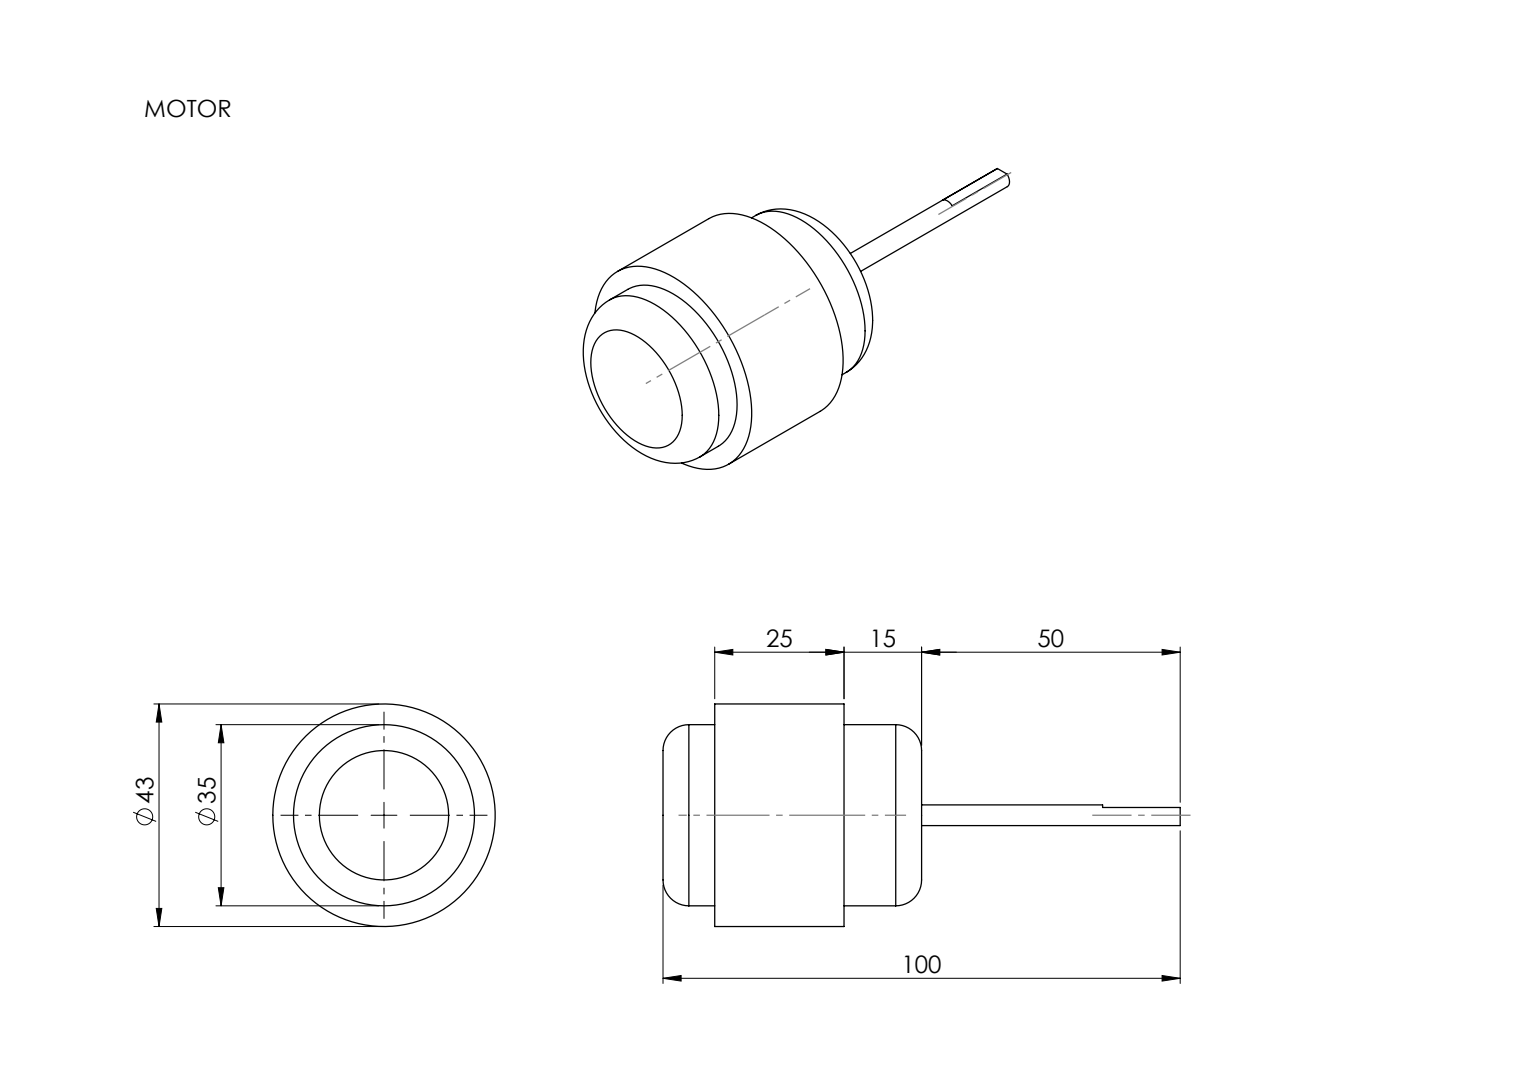
ISO-10303-21;
HEADER;
FILE_DESCRIPTION (('STEP AP214'),
    '1' );
FILE_NAME ('motor.step',
    '2026-10-08T15:02:10',
    ( '' ),
    ( '' ),
    'SwSTEP 2.0',
    'SolidWorks 2026',
    '' );
FILE_SCHEMA (( 'AUTOMOTIVE_DESIGN' ));
ENDSEC;

DATA;
#4=SHAPE_REPRESENTATION_RELATIONSHIP ( 'NONE' , 'NONE' ,  #21505, #10999 ) ;
#67=CARTESIAN_POINT ( 'NONE',  ( 1.322875655532295358, 1.500000000000000000, -105.0000000000000000 ) ) ;
#83=CARTESIAN_POINT ( 'NONE',  ( 12.50000000000000355, 0.000000000000000000, -65.00000000000000000 ) ) ;
#120=CIRCLE ( 'NONE', #7315, 21.50000000000000711 ) ;
#225=AXIS2_PLACEMENT_3D ( 'NONE', #7569, #15900, #3952 ) ;
#288=DIRECTION ( 'NONE',  ( -1.000000000000000000, 0.000000000000000000, 0.000000000000000000 ) ) ;
#339=CARTESIAN_POINT ( 'NONE',  ( 1.322875655532295358, 1.500000000000000000, -120.0000000000000000 ) ) ;
#349=ORIENTED_EDGE ( 'NONE', *, *, #13277, .F. ) ;
#500=CARTESIAN_POINT ( 'NONE',  ( -17.50000000000001066, 2.143131898507869431E-15, -30.00000000000000000 ) ) ;
#540=AXIS2_PLACEMENT_3D ( 'NONE', #11823, #9916, #17115 ) ;
#660=AXIS2_PLACEMENT_3D ( 'NONE', #18313, #757, #9432 ) ;
#665=DIRECTION ( 'NONE',  ( -0.000000000000000000, -0.000000000000000000, -1.000000000000000000 ) ) ;
#686=DIRECTION ( 'NONE',  ( -0.000000000000000000, -0.000000000000000000, -1.000000000000000000 ) ) ;
#711=FACE_OUTER_BOUND ( 'NONE', #8838, .T. ) ;
#756=EDGE_CURVE ( 'NONE', #14896, #1959, #16705, .T. ) ;
#757=DIRECTION ( 'NONE',  ( 0.000000000000000000, 1.000000000000000000, -0.000000000000000000 ) ) ;
#885=CARTESIAN_POINT ( 'NONE',  ( 0.000000000000000000, 0.000000000000000000, -55.00000000000000711 ) ) ;
#907=ORIENTED_EDGE ( 'NONE', *, *, #1716, .T. ) ;
#922=CARTESIAN_POINT ( 'NONE',  ( -21.50000000000000711, 0.000000000000000000, -55.00000000000000711 ) ) ;
#1041=ORIENTED_EDGE ( 'NONE', *, *, #7973, .T. ) ;
#1059=DIRECTION ( 'NONE',  ( -1.000000000000000000, 0.000000000000000000, 0.000000000000000000 ) ) ;
#1102=AXIS2_PLACEMENT_3D ( 'NONE', #16266, #2525, #11420 ) ;
#1133=AXIS2_PLACEMENT_3D ( 'NONE', #4423, #19514, #4101 ) ;
#1161=DIRECTION ( 'NONE',  ( 0.000000000000000000, 0.000000000000000000, 1.000000000000000000 ) ) ;
#1176=PLANE ( 'NONE',  #1102 ) ;
#1275=FACE_OUTER_BOUND ( 'NONE', #18605, .T. ) ;
#1285=CARTESIAN_POINT ( 'NONE',  ( -17.50000000000000355, 2.143131898507868643E-15, -70.00000000000000000 ) ) ;
#1289=CIRCLE ( 'NONE', #225, 21.50000000000000711 ) ;
#1393=ADVANCED_FACE ( 'NONE', ( #19248 ), #3828, .T. ) ;
#1497=AXIS2_PLACEMENT_3D ( 'NONE', #10710, #17575, #21149 ) ;
#1509=EDGE_CURVE ( 'NONE', #11033, #10050, #11370, .T. ) ;
#1518=CARTESIAN_POINT ( 'NONE',  ( -12.50000000000000355, 1.530808498934191916E-15, -25.00000000000000000 ) ) ;
#1534=DIRECTION ( 'NONE',  ( -0.000000000000000000, -0.000000000000000000, -1.000000000000000000 ) ) ;
#1538=CARTESIAN_POINT ( 'NONE',  ( 0.000000000000000000, 0.000000000000000000, -120.0000000000000142 ) ) ;
#1544=AXIS2_PLACEMENT_3D ( 'NONE', #2541, #8986, #15960 ) ;
#1652=( GEOMETRIC_REPRESENTATION_CONTEXT ( 3 ) GLOBAL_UNCERTAINTY_ASSIGNED_CONTEXT ( ( #16412 ) ) GLOBAL_UNIT_ASSIGNED_CONTEXT ( ( #9478, #6196, #11385 ) ) REPRESENTATION_CONTEXT ( 'NONE', 'WORKASPACE' ) );
#1655=DIRECTION ( 'NONE',  ( -1.000000000000000000, 0.000000000000000000, 0.000000000000000000 ) ) ;
#1703=EDGE_LOOP ( 'NONE', ( #10346, #17287, #5811, #6098 ) ) ;
#1716=EDGE_CURVE ( 'NONE', #10973, #3502, #2231, .T. ) ;
#1782=CARTESIAN_POINT ( 'NONE',  ( -17.50000000000000355, 2.143131898507868643E-15, -25.00000000000000000 ) ) ;
#1820=ADVANCED_FACE ( 'NONE', ( #4264 ), #5099, .T. ) ;
#1841=ORIENTED_EDGE ( 'NONE', *, *, #2125, .F. ) ;
#1851=DIRECTION ( 'NONE',  ( 1.000000000000000000, 0.000000000000000000, 0.000000000000000000 ) ) ;
#1889=ORIENTED_EDGE ( 'NONE', *, *, #5608, .T. ) ;
#1954=ORIENTED_EDGE ( 'NONE', *, *, #3358, .F. ) ;
#1959=VERTEX_POINT ( 'NONE', #1782 ) ;
#2125=EDGE_CURVE ( 'NONE', #3502, #10973, #8356, .T. ) ;
#2137=ORIENTED_EDGE ( 'NONE', *, *, #15468, .T. ) ;
#2154=FACE_BOUND ( 'NONE', #18087, .T. ) ;
#2231=CIRCLE ( 'NONE', #4373, 12.50000000000000355 ) ;
#2290=AXIS2_PLACEMENT_3D ( 'NONE', #7537, #2559, #2674 ) ;
#2307=CARTESIAN_POINT ( 'NONE',  ( 17.50000000000000355, 0.000000000000000000, -70.00000000000000000 ) ) ;
#2443=ORIENTED_EDGE ( 'NONE', *, *, #14102, .F. ) ;
#2525=DIRECTION ( 'NONE',  ( 0.000000000000000000, 0.000000000000000000, 1.000000000000000000 ) ) ;
#2541=CARTESIAN_POINT ( 'NONE',  ( 0.000000000000000000, 0.000000000000000000, -70.00000000000000000 ) ) ;
#2559=DIRECTION ( 'NONE',  ( 0.000000000000000000, 0.000000000000000000, -1.000000000000000000 ) ) ;
#2575=DIRECTION ( 'NONE',  ( 0.000000000000000000, 0.000000000000000000, 1.000000000000000000 ) ) ;
#2624=ORIENTED_EDGE ( 'NONE', *, *, #19790, .T. ) ;
#2653=DIRECTION ( 'NONE',  ( -1.000000000000000000, 0.000000000000000000, 0.000000000000000000 ) ) ;
#2674=DIRECTION ( 'NONE',  ( -1.000000000000000000, 0.000000000000000000, 0.000000000000000000 ) ) ;
#2707=DIRECTION ( 'NONE',  ( 1.000000000000000000, 0.000000000000000000, 0.000000000000000000 ) ) ;
#2759=CARTESIAN_POINT ( 'NONE',  ( 0.000000000000000000, 0.000000000000000000, -30.00000000000000000 ) ) ;
#2772=DIRECTION ( 'NONE',  ( 1.000000000000000000, 0.000000000000000000, 0.000000000000000000 ) ) ;
#2801=CIRCLE ( 'NONE', #18270, 17.50000000000001066 ) ;
#2821=AXIS2_PLACEMENT_3D ( 'NONE', #21893, #4675, #16957 ) ;
#2891=DIRECTION ( 'NONE',  ( -0.000000000000000000, -0.000000000000000000, -1.000000000000000000 ) ) ;
#2914=EDGE_CURVE ( 'NONE', #18650, #10973, #5339, .T. ) ;
#2919=AXIS2_PLACEMENT_3D ( 'NONE', #18211, #7637, #2772 ) ;
#2932=VECTOR ( 'NONE', #16594, 1000.000000000000000 ) ;
#2981=ORIENTED_EDGE ( 'NONE', *, *, #8744, .T. ) ;
#3040=VERTEX_POINT ( 'NONE', #16620 ) ;
#3076=MECHANICAL_DESIGN_GEOMETRIC_PRESENTATION_REPRESENTATION('',(#21759),#15681);
#3123=CARTESIAN_POINT ( 'NONE',  ( 0.000000000000000000, 0.000000000000000000, -70.00000000000000000 ) ) ;
#3153=EDGE_LOOP ( 'NONE', ( #14173, #10426, #15370, #5728 ) ) ;
#3180=DIRECTION ( 'NONE',  ( -0.000000000000000000, -0.000000000000000000, -1.000000000000000000 ) ) ;
#3186=ADVANCED_FACE ( 'NONE', ( #16185 ), #18207, .T. ) ;
#3214=DIRECTION ( 'NONE',  ( 1.000000000000000000, 0.000000000000000000, 0.000000000000000000 ) ) ;
#3222=DIRECTION ( 'NONE',  ( -1.000000000000000000, 0.000000000000000000, 0.000000000000000000 ) ) ;
#3358=EDGE_CURVE ( 'NONE', #20674, #9897, #2801, .T. ) ;
#3364=AXIS2_PLACEMENT_3D ( 'NONE', #18542, #13356, #13475 ) ;
#3367=DIRECTION ( 'NONE',  ( -0.000000000000000000, -0.000000000000000000, -1.000000000000000000 ) ) ;
#3437=ORIENTED_EDGE ( 'NONE', *, *, #20358, .F. ) ;
#3438=MECHANICAL_DESIGN_GEOMETRIC_PRESENTATION_REPRESENTATION('',(#17109),#9213);
#3502=VERTEX_POINT ( 'NONE', #9985 ) ;
#3510=CARTESIAN_POINT ( 'NONE',  ( 0.000000000000000000, 0.000000000000000000, -120.0000000000000142 ) ) ;
#3538=ADVANCED_FACE ( 'NONE', ( #22237 ), #13622, .T. ) ;
#3714=LINE ( 'NONE', #4051, #14959 ) ;
#3828=PLANE ( 'NONE',  #1497 ) ;
#3873=VERTEX_POINT ( 'NONE', #67 ) ;
#3879=EDGE_LOOP ( 'NONE', ( #907, #18094 ) ) ;
#3952=DIRECTION ( 'NONE',  ( -1.000000000000000000, 0.000000000000000000, 0.000000000000000000 ) ) ;
#3999=DIRECTION ( 'NONE',  ( -0.000000000000000000, -0.000000000000000000, -1.000000000000000000 ) ) ;
#4051=CARTESIAN_POINT ( 'NONE',  ( -17.50000000000000355, 2.143131898507868643E-15, -70.00000000000000000 ) ) ;
#4073=CIRCLE ( 'NONE', #8401, 5.000000000000004441 ) ;
#4074=FACE_OUTER_BOUND ( 'NONE', #10781, .T. ) ;
#4101=DIRECTION ( 'NONE',  ( 1.000000000000000000, 0.000000000000000000, 0.000000000000000000 ) ) ;
#4185=CARTESIAN_POINT ( 'NONE',  ( -1.322875655532295358, 1.500000000000000000, -378.2244600276337678 ) ) ;
#4205=ORIENTED_EDGE ( 'NONE', *, *, #11174, .F. ) ;
#4264=FACE_OUTER_BOUND ( 'NONE', #16799, .T. ) ;
#4302=LINE ( 'NONE', #4747, #15666 ) ;
#4354=CARTESIAN_POINT ( 'NONE',  ( 0.000000000000000000, 0.000000000000000000, -70.00000000000000000 ) ) ;
#4373=AXIS2_PLACEMENT_3D ( 'NONE', #14970, #4701, #14853 ) ;
#4398=CIRCLE ( 'NONE', #17007, 17.50000000000001066 ) ;
#4423=CARTESIAN_POINT ( 'NONE',  ( 0.000000000000000000, 0.000000000000000000, -70.00000000000000000 ) ) ;
#4469=CARTESIAN_POINT ( 'NONE',  ( 0.000000000000000000, 0.000000000000000000, -105.0000000000000142 ) ) ;
#4499=CARTESIAN_POINT ( 'NONE',  ( 0.000000000000000000, 0.000000000000000000, -70.00000000000000000 ) ) ;
#4512=CARTESIAN_POINT ( 'NONE',  ( 2.000000000000000000, 0.000000000000000000, -120.0000000000000142 ) ) ;
#4528=APPLICATION_CONTEXT ( 'automotive_design' ) ;
#4544=FACE_BOUND ( 'NONE', #13844, .T. ) ;
#4576=ADVANCED_FACE ( 'NONE', ( #7498 ), #14585, .T. ) ;
#4581=CARTESIAN_POINT ( 'NONE',  ( 1.322875655532295358, 1.500000000000000000, -378.2244600276337678 ) ) ;
#4592=ORIENTED_EDGE ( 'NONE', *, *, #6914, .F. ) ;
#4601=EDGE_CURVE ( 'NONE', #11033, #21666, #20906, .T. ) ;
#4675=DIRECTION ( 'NONE',  ( 0.000000000000000000, 0.000000000000000000, 1.000000000000000000 ) ) ;
#4701=DIRECTION ( 'NONE',  ( 0.000000000000000000, 0.000000000000000000, 1.000000000000000000 ) ) ;
#4747=CARTESIAN_POINT ( 'NONE',  ( 21.50000000000001066, 2.632990618166810813E-15, -65.00000000000000000 ) ) ;
#4781=DIRECTION ( 'NONE',  ( -0.000000000000000000, -0.000000000000000000, -1.000000000000000000 ) ) ;
#4838=CARTESIAN_POINT ( 'NONE',  ( 0.000000000000000000, 0.000000000000000000, -30.00000000000000000 ) ) ;
#4919=DIRECTION ( 'NONE',  ( 0.000000000000000000, 0.000000000000000000, -1.000000000000000000 ) ) ;
#4928=EDGE_LOOP ( 'NONE', ( #14011, #17456, #18782, #21763 ) ) ;
#4962=EDGE_CURVE ( 'NONE', #1959, #18650, #20526, .T. ) ;
#4993=ORIENTED_EDGE ( 'NONE', *, *, #12242, .T. ) ;
#5016=ADVANCED_FACE ( 'NONE', ( #8082 ), #9066, .T. ) ;
#5018=FACE_OUTER_BOUND ( 'NONE', #18314, .T. ) ;
#5050=PRODUCT_DEFINITION ( 'UNKNOWN', '', #20347, #14402 ) ;
#5099=TOROIDAL_SURFACE ( 'NONE', #20909, 12.50000000000000355, 5.000000000000000000 ) ;
#5165=AXIS2_PLACEMENT_3D ( 'NONE', #19638, #17970, #9201 ) ;
#5180=CARTESIAN_POINT ( 'NONE',  ( -12.50000000000000355, 1.530808498934191916E-15, -65.00000000000000000 ) ) ;
#5198=CIRCLE ( 'NONE', #540, 17.50000000000000355 ) ;
#5339=CIRCLE ( 'NONE', #13989, 5.000000000000000888 ) ;
#5369=DIRECTION ( 'NONE',  ( 0.000000000000000000, 0.000000000000000000, 1.000000000000000000 ) ) ;
#5498=DIRECTION ( 'NONE',  ( -0.000000000000000000, -0.000000000000000000, 1.000000000000000000 ) ) ;
#5545=ADVANCED_FACE ( 'NONE', ( #5018 ), #6604, .T. ) ;
#5550=ORIENTED_EDGE ( 'NONE', *, *, #17171, .F. ) ;
#5552=ORIENTED_EDGE ( 'NONE', *, *, #15025, .F. ) ;
#5608=EDGE_CURVE ( 'NONE', #7196, #9986, #6530, .T. ) ;
#5692=CARTESIAN_POINT ( 'NONE',  ( -1.322875655532295136, 1.500000000000000000, -120.0000000000000142 ) ) ;
#5728=ORIENTED_EDGE ( 'NONE', *, *, #2914, .F. ) ;
#5750=( NAMED_UNIT ( * ) PLANE_ANGLE_UNIT ( ) SI_UNIT ( $, .RADIAN. ) );
#5781=EDGE_LOOP ( 'NONE', ( #20629, #3437, #20188, #5552 ) ) ;
#5811=ORIENTED_EDGE ( 'NONE', *, *, #6066, .T. ) ;
#5833=DIRECTION ( 'NONE',  ( 1.000000000000000000, 0.000000000000000000, 0.000000000000000000 ) ) ;
#6066=EDGE_CURVE ( 'NONE', #13719, #18650, #19408, .T. ) ;
#6098=ORIENTED_EDGE ( 'NONE', *, *, #13277, .T. ) ;
#6180=ADVANCED_FACE ( 'NONE', ( #4544, #18180 ), #1176, .F. ) ;
#6181=AXIS2_PLACEMENT_3D ( 'NONE', #14396, #5369, #21015 ) ;
#6194=CIRCLE ( 'NONE', #10881, 2.000000000000000000 ) ;
#6196=( NAMED_UNIT ( * ) PLANE_ANGLE_UNIT ( ) SI_UNIT ( $, .RADIAN. ) );
#6203=CARTESIAN_POINT ( 'NONE',  ( 17.50000000000001066, 0.000000000000000000, -55.00000000000000711 ) ) ;
#6225=AXIS2_PLACEMENT_3D ( 'NONE', #11498, #16348, #19926 ) ;
#6287=ORIENTED_EDGE ( 'NONE', *, *, #17683, .F. ) ;
#6414=DIRECTION ( 'NONE',  ( 1.000000000000000000, 0.000000000000000000, 0.000000000000000000 ) ) ;
#6454=EDGE_CURVE ( 'NONE', #14043, #20674, #3714, .T. ) ;
#6524=CARTESIAN_POINT ( 'NONE',  ( 17.50000000000000355, 0.000000000000000000, -25.00000000000000000 ) ) ;
#6530=CIRCLE ( 'NONE', #9416, 2.000000000000000000 ) ;
#6532=( NAMED_UNIT ( * ) SI_UNIT ( $, .STERADIAN. ) SOLID_ANGLE_UNIT ( ) );
#6604=CYLINDRICAL_SURFACE ( 'NONE', #19110, 17.50000000000000355 ) ;
#6650=PRESENTATION_STYLE_ASSIGNMENT (( #18694 ) ) ;
#6669=ORIENTED_EDGE ( 'NONE', *, *, #13487, .T. ) ;
#6677=AXIS2_PLACEMENT_3D ( 'NONE', #18028, #16226, #2707 ) ;
#6692=COLOUR_RGB ( '', 0.66274510, 0.83137255, 0.94901961) ;
#6748=ORIENTED_EDGE ( 'NONE', *, *, #756, .T. ) ;
#6764=( LENGTH_UNIT ( ) NAMED_UNIT ( * ) SI_UNIT ( .MILLI., .METRE. ) );
#6914=EDGE_CURVE ( 'NONE', #9939, #9897, #16068, .T. ) ;
#7196=VERTEX_POINT ( 'NONE', #19369 ) ;
#7207=DIRECTION ( 'NONE',  ( -1.000000000000000000, 0.000000000000000000, 0.000000000000000000 ) ) ;
#7261=VECTOR ( 'NONE', #10925, 1000.000000000000000 ) ;
#7291=DIRECTION ( 'NONE',  ( 1.000000000000000000, 0.000000000000000000, 0.000000000000000000 ) ) ;
#7315=AXIS2_PLACEMENT_3D ( 'NONE', #885, #665, #16199 ) ;
#7318=CARTESIAN_POINT ( 'NONE',  ( 0.000000000000000000, 0.000000000000000000, -120.0000000000000142 ) ) ;
#7335=ADVANCED_FACE ( 'NONE', ( #12628, #2154 ), #9034, .F. ) ;
#7352=DIRECTION ( 'NONE',  ( -0.000000000000000000, 0.000000000000000000, -1.000000000000000000 ) ) ;
#7376=AXIS2_PLACEMENT_3D ( 'NONE', #1518, #20408, #8723 ) ;
#7396=AXIS2_PLACEMENT_3D ( 'NONE', #15532, #3367, #10249 ) ;
#7414=VECTOR ( 'NONE', #17361, 1000.000000000000000 ) ;
#7421=ORIENTED_EDGE ( 'NONE', *, *, #8542, .F. ) ;
#7498=FACE_OUTER_BOUND ( 'NONE', #1703, .T. ) ;
#7537=CARTESIAN_POINT ( 'NONE',  ( 0.000000000000000000, 0.000000000000000000, -105.0000000000000142 ) ) ;
#7540=DIRECTION ( 'NONE',  ( 0.000000000000000000, 0.000000000000000000, 1.000000000000000000 ) ) ;
#7569=CARTESIAN_POINT ( 'NONE',  ( 0.000000000000000000, 0.000000000000000000, -55.00000000000000711 ) ) ;
#7612=ORIENTED_EDGE ( 'NONE', *, *, #3358, .T. ) ;
#7637=DIRECTION ( 'NONE',  ( 0.000000000000000000, 0.000000000000000000, 1.000000000000000000 ) ) ;
#7673=AXIS2_PLACEMENT_3D ( 'NONE', #9084, #3999, #7291 ) ;
#7728=DIRECTION ( 'NONE',  ( -0.000000000000000000, -0.000000000000000000, -1.000000000000000000 ) ) ;
#7862=UNCERTAINTY_MEASURE_WITH_UNIT (LENGTH_MEASURE( 1.000000000000000082E-05 ), #6764, 'distance_accuracy_value', 'NONE');
#7942=ORIENTED_EDGE ( 'NONE', *, *, #9134, .T. ) ;
#7973=EDGE_CURVE ( 'NONE', #14896, #13719, #8140, .T. ) ;
#8042=AXIS2_PLACEMENT_3D ( 'NONE', #7318, #5498, #19229 ) ;
#8082=FACE_OUTER_BOUND ( 'NONE', #5781, .T. ) ;
#8131=VECTOR ( 'NONE', #21323, 1000.000000000000000 ) ;
#8140=CIRCLE ( 'NONE', #20705, 17.50000000000001066 ) ;
#8159=DIRECTION ( 'NONE',  ( 0.000000000000000000, 0.000000000000000000, 1.000000000000000000 ) ) ;
#8297=APPLICATION_CONTEXT ( 'automotive_design' ) ;
#8350=VERTEX_POINT ( 'NONE', #17645 ) ;
#8356=CIRCLE ( 'NONE', #6181, 12.50000000000000355 ) ;
#8385=DIRECTION ( 'NONE',  ( 0.000000000000000000, 0.000000000000000000, -1.000000000000000000 ) ) ;
#8396=CARTESIAN_POINT ( 'NONE',  ( -2.000000000000000000, 2.449293598294706414E-16, -120.0000000000000142 ) ) ;
#8401=AXIS2_PLACEMENT_3D ( 'NONE', #83, #12016, #4919 ) ;
#8416=DIRECTION ( 'NONE',  ( 0.000000000000000000, 0.000000000000000000, -1.000000000000000000 ) ) ;
#8449=ADVANCED_FACE ( 'NONE', ( #12579, #17871 ), #19422, .F. ) ;
#8482=ORIENTED_EDGE ( 'NONE', *, *, #4601, .T. ) ;
#8534=PRODUCT_DEFINITION_SHAPE ( 'NONE', 'NONE',  #5050 ) ;
#8542=EDGE_CURVE ( 'NONE', #14013, #9212, #19535, .T. ) ;
#8598=FACE_OUTER_BOUND ( 'NONE', #19239, .T. ) ;
#8691=ORIENTED_EDGE ( 'NONE', *, *, #21072, .T. ) ;
#8723=DIRECTION ( 'NONE',  ( -1.000000000000000000, 1.224646799147353454E-16, 0.000000000000000000 ) ) ;
#8735=CIRCLE ( 'NONE', #17733, 12.50000000000000355 ) ;
#8744=EDGE_CURVE ( 'NONE', #13719, #14896, #4398, .T. ) ;
#8783=EDGE_CURVE ( 'NONE', #21666, #11033, #11954, .T. ) ;
#8789=CIRCLE ( 'NONE', #18130, 17.50000000000000355 ) ;
#8838=EDGE_LOOP ( 'NONE', ( #4205, #13568, #21735, #16900, #15673, #4993, #9825, #16082 ) ) ;
#8874=CARTESIAN_POINT ( 'NONE',  ( 2.000000000000000000, 0.000000000000000000, -70.00000000000000000 ) ) ;
#8986=DIRECTION ( 'NONE',  ( 0.000000000000000000, 0.000000000000000000, 1.000000000000000000 ) ) ;
#9034=PLANE ( 'NONE',  #12451 ) ;
#9066=TOROIDAL_SURFACE ( 'NONE', #2919, 12.50000000000000355, 5.000000000000000000 ) ;
#9084=CARTESIAN_POINT ( 'NONE',  ( 0.000000000000000000, 0.000000000000000000, -70.00000000000000000 ) ) ;
#9096=ORIENTED_EDGE ( 'NONE', *, *, #7973, .F. ) ;
#9127=ORIENTED_EDGE ( 'NONE', *, *, #2914, .T. ) ;
#9134=EDGE_CURVE ( 'NONE', #9986, #14013, #18790, .T. ) ;
#9178=CARTESIAN_POINT ( 'NONE',  ( -17.50000000000001066, 2.143131898507869431E-15, -55.00000000000000711 ) ) ;
#9201=DIRECTION ( 'NONE',  ( 1.000000000000000000, 0.000000000000000000, 0.000000000000000000 ) ) ;
#9212=VERTEX_POINT ( 'NONE', #19049 ) ;
#9213=( GEOMETRIC_REPRESENTATION_CONTEXT ( 3 ) GLOBAL_UNCERTAINTY_ASSIGNED_CONTEXT ( ( #7862 ) ) GLOBAL_UNIT_ASSIGNED_CONTEXT ( ( #6764, #15434, #6532 ) ) REPRESENTATION_CONTEXT ( 'NONE', 'WORKASPACE' ) );
#9260=ADVANCED_FACE ( 'NONE', ( #4074 ), #15801, .T. ) ;
#9320=ORIENTED_EDGE ( 'NONE', *, *, #22019, .F. ) ;
#9360=ORIENTED_EDGE ( 'NONE', *, *, #4962, .T. ) ;
#9393=ORIENTED_EDGE ( 'NONE', *, *, #1509, .F. ) ;
#9403=EDGE_CURVE ( 'NONE', #13305, #8350, #21065, .T. ) ;
#9416=AXIS2_PLACEMENT_3D ( 'NONE', #1538, #8416, #1655 ) ;
#9432=DIRECTION ( 'NONE',  ( 0.000000000000000000, 0.000000000000000000, 1.000000000000000000 ) ) ;
#9448=FACE_OUTER_BOUND ( 'NONE', #15163, .T. ) ;
#9478=( LENGTH_UNIT ( ) NAMED_UNIT ( * ) SI_UNIT ( .MILLI., .METRE. ) );
#9485=VECTOR ( 'NONE', #11457, 1000.000000000000000 ) ;
#9486=CYLINDRICAL_SURFACE ( 'NONE', #6225, 21.50000000000001066 ) ;
#9655=CARTESIAN_POINT ( 'NONE',  ( 12.50000000000000355, 0.000000000000000000, -20.00000000000000000 ) ) ;
#9737=ORIENTED_EDGE ( 'NONE', *, *, #6454, .F. ) ;
#9803=AXIS2_PLACEMENT_3D ( 'NONE', #12905, #4781, #2653 ) ;
#9825=ORIENTED_EDGE ( 'NONE', *, *, #12429, .F. ) ;
#9870=ORIENTED_EDGE ( 'NONE', *, *, #20358, .T. ) ;
#9897=VERTEX_POINT ( 'NONE', #6203 ) ;
#9916=DIRECTION ( 'NONE',  ( 0.000000000000000000, 0.000000000000000000, 1.000000000000000000 ) ) ;
#9939=VERTEX_POINT ( 'NONE', #19811 ) ;
#9983=ADVANCED_FACE ( 'NONE', ( #14885 ), #9486, .T. ) ;
#9985=CARTESIAN_POINT ( 'NONE',  ( -12.50000000000000355, 1.836970198721030378E-15, -20.00000000000000000 ) ) ;
#9986=VERTEX_POINT ( 'NONE', #4512 ) ;
#10050=VERTEX_POINT ( 'NONE', #922 ) ;
#10066=CARTESIAN_POINT ( 'NONE',  ( 0.000000000000000000, 0.000000000000000000, -120.0000000000000142 ) ) ;
#10120=ORIENTED_EDGE ( 'NONE', *, *, #10180, .T. ) ;
#10124=ORIENTED_EDGE ( 'NONE', *, *, #21072, .F. ) ;
#10153=DIRECTION ( 'NONE',  ( 1.224646799147353207E-16, 1.000000000000000000, -0.000000000000000000 ) ) ;
#10180=EDGE_CURVE ( 'NONE', #3040, #14043, #14854, .T. ) ;
#10249=DIRECTION ( 'NONE',  ( -1.000000000000000000, 0.000000000000000000, 0.000000000000000000 ) ) ;
#10346=ORIENTED_EDGE ( 'NONE', *, *, #756, .F. ) ;
#10367=ORIENTED_EDGE ( 'NONE', *, *, #15468, .F. ) ;
#10390=DIRECTION ( 'NONE',  ( 0.000000000000000000, 0.000000000000000000, -1.000000000000000000 ) ) ;
#10416=CYLINDRICAL_SURFACE ( 'NONE', #11251, 21.50000000000001066 ) ;
#10426=ORIENTED_EDGE ( 'NONE', *, *, #14102, .T. ) ;
#10548=VECTOR ( 'NONE', #3222, 1000.000000000000000 ) ;
#10556=DIRECTION ( 'NONE',  ( -1.000000000000000000, 0.000000000000000000, 0.000000000000000000 ) ) ;
#10610=DIRECTION ( 'NONE',  ( -1.000000000000000000, 0.000000000000000000, -0.000000000000000000 ) ) ;
#10685=EDGE_LOOP ( 'NONE', ( #9870, #19241 ) ) ;
#10710=CARTESIAN_POINT ( 'NONE',  ( 0.000000000000000000, 0.000000000000000000, -20.00000000000000000 ) ) ;
#10724=PRESENTATION_STYLE_ASSIGNMENT (( #17813 ) ) ;
#10740=ORIENTED_EDGE ( 'NONE', *, *, #13487, .F. ) ;
#10781=EDGE_LOOP ( 'NONE', ( #9737, #19755, #12772, #2137 ) ) ;
#10881=AXIS2_PLACEMENT_3D ( 'NONE', #4499, #686, #14429 ) ;
#10925=DIRECTION ( 'NONE',  ( -0.000000000000000000, -0.000000000000000000, -1.000000000000000000 ) ) ;
#10927=AXIS2_PLACEMENT_3D ( 'NONE', #4469, #11350, #18220 ) ;
#10973=VERTEX_POINT ( 'NONE', #9655 ) ;
#10979=CARTESIAN_POINT ( 'NONE',  ( 0.000000000000000000, 0.000000000000000000, -30.00000000000000000 ) ) ;
#10999=ADVANCED_BREP_SHAPE_REPRESENTATION ( '', ( #22038, #6677 ), #1652 ) ;
#11013=ORIENTED_EDGE ( 'NONE', *, *, #16421, .F. ) ;
#11025=CARTESIAN_POINT ( 'NONE',  ( 12.50000000000000355, 0.000000000000000000, -70.00000000000000000 ) ) ;
#11033=VERTEX_POINT ( 'NONE', #18319 ) ;
#11174=EDGE_CURVE ( 'NONE', #14013, #13305, #16660, .T. ) ;
#11177=EDGE_LOOP ( 'NONE', ( #17966, #13696 ) ) ;
#11250=CARTESIAN_POINT ( 'NONE',  ( 0.000000000000000000, 0.000000000000000000, -65.00000000000000000 ) ) ;
#11251=AXIS2_PLACEMENT_3D ( 'NONE', #15075, #19067, #288 ) ;
#11330=EDGE_LOOP ( 'NONE', ( #7421, #18893, #17633, #15312 ) ) ;
#11350=DIRECTION ( 'NONE',  ( 0.000000000000000000, 0.000000000000000000, -1.000000000000000000 ) ) ;
#11370=LINE ( 'NONE', #17907, #7261 ) ;
#11385=( NAMED_UNIT ( * ) SI_UNIT ( $, .STERADIAN. ) SOLID_ANGLE_UNIT ( ) );
#11398=EDGE_LOOP ( 'NONE', ( #10124, #17672, #19566, #9320 ) ) ;
#11420=DIRECTION ( 'NONE',  ( 1.000000000000000000, 0.000000000000000000, -0.000000000000000000 ) ) ;
#11429=CARTESIAN_POINT ( 'NONE',  ( -17.50000000000000355, 2.143131898507868643E-15, -65.00000000000000000 ) ) ;
#11457=DIRECTION ( 'NONE',  ( 0.000000000000000000, 0.000000000000000000, 1.000000000000000000 ) ) ;
#11498=CARTESIAN_POINT ( 'NONE',  ( 0.000000000000000000, 0.000000000000000000, -65.00000000000000000 ) ) ;
#11557=DIRECTION ( 'NONE',  ( 0.000000000000000000, 0.000000000000000000, 1.000000000000000000 ) ) ;
#11568=FACE_OUTER_BOUND ( 'NONE', #11398, .T. ) ;
#11714=DIRECTION ( 'NONE',  ( -0.000000000000000000, -0.000000000000000000, -1.000000000000000000 ) ) ;
#11787=CARTESIAN_POINT ( 'NONE',  ( 0.000000000000000000, 0.000000000000000000, -70.00000000000000000 ) ) ;
#11823=CARTESIAN_POINT ( 'NONE',  ( 0.000000000000000000, 0.000000000000000000, -65.00000000000000000 ) ) ;
#11879=EDGE_CURVE ( 'NONE', #7196, #13305, #15977, .T. ) ;
#11908=ADVANCED_FACE ( 'NONE', ( #14188 ), #14073, .T. ) ;
#11926=VECTOR ( 'NONE', #8159, 1000.000000000000000 ) ;
#11954=CIRCLE ( 'NONE', #9803, 21.50000000000001066 ) ;
#11989=VECTOR ( 'NONE', #7207, 1000.000000000000000 ) ;
#11997=ORIENTED_EDGE ( 'NONE', *, *, #17120, .T. ) ;
#12009=CIRCLE ( 'NONE', #2290, 2.000000000000000000 ) ;
#12016=DIRECTION ( 'NONE',  ( 0.000000000000000000, -1.000000000000000000, 0.000000000000000000 ) ) ;
#12030=CIRCLE ( 'NONE', #7376, 5.000000000000000888 ) ;
#12079=PLANE ( 'NONE',  #20689 ) ;
#12174=CLOSED_SHELL ( 'NONE', ( #5545, #3538, #9983, #14561, #1820, #21092, #9260, #8449, #5016, #11908, #21845, #3186, #12520, #7335, #20015, #6180, #1393, #16205, #4576 ) ) ;
#12242=EDGE_CURVE ( 'NONE', #7196, #3873, #12820, .T. ) ;
#12296=( LENGTH_UNIT ( ) NAMED_UNIT ( * ) SI_UNIT ( .MILLI., .METRE. ) );
#12304=DIRECTION ( 'NONE',  ( 1.000000000000000000, 0.000000000000000000, 0.000000000000000000 ) ) ;
#12412=FILL_AREA_STYLE ('',( #14109 ) ) ;
#12429=EDGE_CURVE ( 'NONE', #8350, #3873, #12009, .T. ) ;
#12451=AXIS2_PLACEMENT_3D ( 'NONE', #15898, #7352, #21054 ) ;
#12520=ADVANCED_FACE ( 'NONE', ( #16418 ), #21684, .T. ) ;
#12530=DIRECTION ( 'NONE',  ( 0.000000000000000000, 0.000000000000000000, 1.000000000000000000 ) ) ;
#12579=FACE_BOUND ( 'NONE', #15188, .T. ) ;
#12628=FACE_OUTER_BOUND ( 'NONE', #11177, .T. ) ;
#12630=( NAMED_UNIT ( * ) SI_UNIT ( $, .STERADIAN. ) SOLID_ANGLE_UNIT ( ) );
#12673=PRODUCT_CONTEXT ( 'NONE', #4528, 'mechanical' ) ;
#12772=ORIENTED_EDGE ( 'NONE', *, *, #6914, .T. ) ;
#12820=LINE ( 'NONE', #4581, #9485 ) ;
#12905=CARTESIAN_POINT ( 'NONE',  ( 0.000000000000000000, 0.000000000000000000, -30.00000000000000000 ) ) ;
#13050=VECTOR ( 'NONE', #14493, 1000.000000000000000 ) ;
#13277=EDGE_CURVE ( 'NONE', #18650, #1959, #8789, .T. ) ;
#13295=ORIENTED_EDGE ( 'NONE', *, *, #11879, .F. ) ;
#13305=VERTEX_POINT ( 'NONE', #5692 ) ;
#13313=DIRECTION ( 'NONE',  ( 1.000000000000000000, 0.000000000000000000, 0.000000000000000000 ) ) ;
#13343=DIRECTION ( 'NONE',  ( -0.000000000000000000, -0.000000000000000000, -1.000000000000000000 ) ) ;
#13356=DIRECTION ( 'NONE',  ( 0.000000000000000000, 0.000000000000000000, -1.000000000000000000 ) ) ;
#13398=VECTOR ( 'NONE', #12530, 1000.000000000000000 ) ;
#13475=DIRECTION ( 'NONE',  ( -1.000000000000000000, 0.000000000000000000, 0.000000000000000000 ) ) ;
#13487=EDGE_CURVE ( 'NONE', #9939, #14043, #14889, .T. ) ;
#13551=CARTESIAN_POINT ( 'NONE',  ( 21.50000000000001066, 2.632990618166810813E-15, -30.00000000000000000 ) ) ;
#13559=CARTESIAN_POINT ( 'NONE',  ( 0.000000000000000000, 0.000000000000000000, -25.00000000000000000 ) ) ;
#13568=ORIENTED_EDGE ( 'NONE', *, *, #8542, .T. ) ;
#13622=TOROIDAL_SURFACE ( 'NONE', #2821, 12.50000000000000355, 5.000000000000000000 ) ;
#13696=ORIENTED_EDGE ( 'NONE', *, *, #8783, .F. ) ;
#13719=VERTEX_POINT ( 'NONE', #21653 ) ;
#13745=SURFACE_SIDE_STYLE ('',( #20359 ) ) ;
#13841=AXIS2_PLACEMENT_3D ( 'NONE', #21824, #16664, #6414 ) ;
#13844=EDGE_LOOP ( 'NONE', ( #10367, #1954 ) ) ;
#13936=LINE ( 'NONE', #15401, #10548 ) ;
#13978=DIRECTION ( 'NONE',  ( 1.000000000000000000, 0.000000000000000000, 0.000000000000000000 ) ) ;
#13989=AXIS2_PLACEMENT_3D ( 'NONE', #19653, #16404, #14827 ) ;
#14011=ORIENTED_EDGE ( 'NONE', *, *, #12242, .F. ) ;
#14013=VERTEX_POINT ( 'NONE', #8396 ) ;
#14043=VERTEX_POINT ( 'NONE', #11429 ) ;
#14073=CYLINDRICAL_SURFACE ( 'NONE', #8042, 2.000000000000000000 ) ;
#14102=EDGE_CURVE ( 'NONE', #1959, #3502, #12030, .T. ) ;
#14109=FILL_AREA_STYLE_COLOUR ( '', #6692 ) ;
#14173=ORIENTED_EDGE ( 'NONE', *, *, #4962, .F. ) ;
#14188=FACE_OUTER_BOUND ( 'NONE', #11330, .T. ) ;
#14230=CARTESIAN_POINT ( 'NONE',  ( 0.000000000000000000, 0.000000000000000000, -70.00000000000000000 ) ) ;
#14239=COLOUR_RGB ( '', 0.66274510, 0.83137255, 0.94901961) ;
#14375=EDGE_LOOP ( 'NONE', ( #8482, #8691, #14397, #9393 ) ) ;
#14382=CARTESIAN_POINT ( 'NONE',  ( 17.50000000000000355, 0.000000000000000000, -70.00000000000000000 ) ) ;
#14396=CARTESIAN_POINT ( 'NONE',  ( 0.000000000000000000, 0.000000000000000000, -20.00000000000000000 ) ) ;
#14397=ORIENTED_EDGE ( 'NONE', *, *, #19790, .F. ) ;
#14402=PRODUCT_DEFINITION_CONTEXT ( 'detailed design', #8297, 'design' ) ;
#14429=DIRECTION ( 'NONE',  ( 1.000000000000000000, 0.000000000000000000, 0.000000000000000000 ) ) ;
#14493=DIRECTION ( 'NONE',  ( -0.000000000000000000, -0.000000000000000000, 1.000000000000000000 ) ) ;
#14561=ADVANCED_FACE ( 'NONE', ( #711 ), #16139, .T. ) ;
#14585=CYLINDRICAL_SURFACE ( 'NONE', #1133, 17.50000000000000355 ) ;
#14591=AXIS2_PLACEMENT_3D ( 'NONE', #21744, #1161, #13313 ) ;
#14744=DIRECTION ( 'NONE',  ( 1.000000000000000000, 0.000000000000000000, 0.000000000000000000 ) ) ;
#14827=DIRECTION ( 'NONE',  ( 0.000000000000000000, 0.000000000000000000, -1.000000000000000000 ) ) ;
#14853=DIRECTION ( 'NONE',  ( 1.000000000000000000, 0.000000000000000000, 0.000000000000000000 ) ) ;
#14854=CIRCLE ( 'NONE', #17731, 5.000000000000000888 ) ;
#14885=FACE_OUTER_BOUND ( 'NONE', #14375, .T. ) ;
#14889=CIRCLE ( 'NONE', #5165, 17.50000000000000355 ) ;
#14896=VERTEX_POINT ( 'NONE', #500 ) ;
#14903=CYLINDRICAL_SURFACE ( 'NONE', #14591, 17.50000000000000355 ) ;
#14945=CIRCLE ( 'NONE', #7396, 17.50000000000001066 ) ;
#14959=VECTOR ( 'NONE', #11557, 1000.000000000000000 ) ;
#14970=CARTESIAN_POINT ( 'NONE',  ( 0.000000000000000000, 0.000000000000000000, -20.00000000000000000 ) ) ;
#15025=EDGE_CURVE ( 'NONE', #14043, #9939, #5198, .T. ) ;
#15075=CARTESIAN_POINT ( 'NONE',  ( 0.000000000000000000, 0.000000000000000000, -65.00000000000000000 ) ) ;
#15163=EDGE_LOOP ( 'NONE', ( #2443, #349, #9127, #1841 ) ) ;
#15188=EDGE_LOOP ( 'NONE', ( #11013, #20923 ) ) ;
#15312=ORIENTED_EDGE ( 'NONE', *, *, #16421, .T. ) ;
#15370=ORIENTED_EDGE ( 'NONE', *, *, #1716, .F. ) ;
#15401=CARTESIAN_POINT ( 'NONE',  ( 1.322875655532295358, 1.500000000000000000, -104.9999999999999858 ) ) ;
#15416=ORIENTED_EDGE ( 'NONE', *, *, #6454, .T. ) ;
#15434=( NAMED_UNIT ( * ) PLANE_ANGLE_UNIT ( ) SI_UNIT ( $, .RADIAN. ) );
#15468=EDGE_CURVE ( 'NONE', #9897, #20674, #14945, .T. ) ;
#15532=CARTESIAN_POINT ( 'NONE',  ( 0.000000000000000000, 0.000000000000000000, -55.00000000000000711 ) ) ;
#15646=TOROIDAL_SURFACE ( 'NONE', #17446, 12.50000000000000355, 5.000000000000000000 ) ;
#15666=VECTOR ( 'NONE', #20154, 1000.000000000000000 ) ;
#15673=ORIENTED_EDGE ( 'NONE', *, *, #5608, .F. ) ;
#15681=( GEOMETRIC_REPRESENTATION_CONTEXT ( 3 ) GLOBAL_UNCERTAINTY_ASSIGNED_CONTEXT ( ( #20200 ) ) GLOBAL_UNIT_ASSIGNED_CONTEXT ( ( #12296, #5750, #12630 ) ) REPRESENTATION_CONTEXT ( 'NONE', 'WORKASPACE' ) );
#15801=CYLINDRICAL_SURFACE ( 'NONE', #18432, 17.50000000000000355 ) ;
#15898=CARTESIAN_POINT ( 'NONE',  ( 0.000000000000000000, -17.50000000000001066, -30.00000000000000000 ) ) ;
#15900=DIRECTION ( 'NONE',  ( -0.000000000000000000, -0.000000000000000000, -1.000000000000000000 ) ) ;
#15960=DIRECTION ( 'NONE',  ( 1.000000000000000000, 0.000000000000000000, -0.000000000000000000 ) ) ;
#15977=LINE ( 'NONE', #339, #11989 ) ;
#16065=CARTESIAN_POINT ( 'NONE',  ( 0.000000000000000000, 0.000000000000000000, -25.00000000000000000 ) ) ;
#16068=LINE ( 'NONE', #14382, #8131 ) ;
#16082=ORIENTED_EDGE ( 'NONE', *, *, #9403, .F. ) ;
#16139=CYLINDRICAL_SURFACE ( 'NONE', #13841, 2.000000000000000000 ) ;
#16185=FACE_OUTER_BOUND ( 'NONE', #4928, .T. ) ;
#16199=DIRECTION ( 'NONE',  ( -1.000000000000000000, 0.000000000000000000, 0.000000000000000000 ) ) ;
#16205=ADVANCED_FACE ( 'NONE', ( #9448 ), #15646, .T. ) ;
#16226=DIRECTION ( 'NONE',  ( 0.000000000000000000, 0.000000000000000000, 1.000000000000000000 ) ) ;
#16266=CARTESIAN_POINT ( 'NONE',  ( 0.000000000000000000, -17.50000000000001066, -55.00000000000000711 ) ) ;
#16308=DIRECTION ( 'NONE',  ( 1.000000000000000000, 0.000000000000000000, 0.000000000000000000 ) ) ;
#16348=DIRECTION ( 'NONE',  ( -0.000000000000000000, -0.000000000000000000, -1.000000000000000000 ) ) ;
#16402=VERTEX_POINT ( 'NONE', #11025 ) ;
#16404=DIRECTION ( 'NONE',  ( 0.000000000000000000, -1.000000000000000000, 0.000000000000000000 ) ) ;
#16412=UNCERTAINTY_MEASURE_WITH_UNIT (LENGTH_MEASURE( 1.000000000000000082E-05 ), #9478, 'distance_accuracy_value', 'NONE');
#16418=FACE_OUTER_BOUND ( 'NONE', #17266, .T. ) ;
#16421=EDGE_CURVE ( 'NONE', #16736, #9212, #18884, .T. ) ;
#16591=AXIS2_PLACEMENT_3D ( 'NONE', #13559, #3180, #13978 ) ;
#16594=DIRECTION ( 'NONE',  ( 0.000000000000000000, 0.000000000000000000, 1.000000000000000000 ) ) ;
#16620=CARTESIAN_POINT ( 'NONE',  ( -12.50000000000000355, 1.836970198721030378E-15, -70.00000000000000000 ) ) ;
#16660=CIRCLE ( 'NONE', #3364, 2.000000000000000000 ) ;
#16664=DIRECTION ( 'NONE',  ( -0.000000000000000000, -0.000000000000000000, 1.000000000000000000 ) ) ;
#16705=LINE ( 'NONE', #1285, #11926 ) ;
#16736=VERTEX_POINT ( 'NONE', #8874 ) ;
#16799=EDGE_LOOP ( 'NONE', ( #6287, #10120, #10740, #5550 ) ) ;
#16900=ORIENTED_EDGE ( 'NONE', *, *, #21888, .F. ) ;
#16957=DIRECTION ( 'NONE',  ( 1.000000000000000000, 0.000000000000000000, 0.000000000000000000 ) ) ;
#17007=AXIS2_PLACEMENT_3D ( 'NONE', #2759, #13343, #21548 ) ;
#17109=STYLED_ITEM ( 'NONE', ( #6650 ), #10999 ) ;
#17115=DIRECTION ( 'NONE',  ( 1.000000000000000000, 0.000000000000000000, 0.000000000000000000 ) ) ;
#17120=EDGE_CURVE ( 'NONE', #3873, #8350, #13936, .T. ) ;
#17171=EDGE_CURVE ( 'NONE', #16402, #9939, #4073, .T. ) ;
#17266=EDGE_LOOP ( 'NONE', ( #11997, #20742 ) ) ;
#17287=ORIENTED_EDGE ( 'NONE', *, *, #8744, .F. ) ;
#17361=DIRECTION ( 'NONE',  ( -0.000000000000000000, -0.000000000000000000, 1.000000000000000000 ) ) ;
#17369=CIRCLE ( 'NONE', #7673, 12.50000000000000355 ) ;
#17446=AXIS2_PLACEMENT_3D ( 'NONE', #21574, #7540, #16308 ) ;
#17456=ORIENTED_EDGE ( 'NONE', *, *, #11879, .T. ) ;
#17481=CARTESIAN_POINT ( 'NONE',  ( 2.000000000000000000, 0.000000000000000000, -120.0000000000000142 ) ) ;
#17575=DIRECTION ( 'NONE',  ( 0.000000000000000000, 0.000000000000000000, 1.000000000000000000 ) ) ;
#17633=ORIENTED_EDGE ( 'NONE', *, *, #21888, .T. ) ;
#17645=CARTESIAN_POINT ( 'NONE',  ( -1.322875655532295136, 1.500000000000000000, -105.0000000000000142 ) ) ;
#17672=ORIENTED_EDGE ( 'NONE', *, *, #8783, .T. ) ;
#17676=AXIS2_PLACEMENT_3D ( 'NONE', #10979, #17850, #1059 ) ;
#17683=EDGE_CURVE ( 'NONE', #3040, #16402, #17369, .T. ) ;
#17731=AXIS2_PLACEMENT_3D ( 'NONE', #5180, #10153, #19026 ) ;
#17733=AXIS2_PLACEMENT_3D ( 'NONE', #3123, #2891, #1851 ) ;
#17813=SURFACE_STYLE_USAGE ( .BOTH. , #19264 ) ;
#17822=DIRECTION ( 'NONE',  ( 0.000000000000000000, 0.000000000000000000, 1.000000000000000000 ) ) ;
#17850=DIRECTION ( 'NONE',  ( -0.000000000000000000, -0.000000000000000000, -1.000000000000000000 ) ) ;
#17871=FACE_OUTER_BOUND ( 'NONE', #10685, .T. ) ;
#17907=CARTESIAN_POINT ( 'NONE',  ( -21.50000000000001066, 0.000000000000000000, -65.00000000000000000 ) ) ;
#17966=ORIENTED_EDGE ( 'NONE', *, *, #4601, .F. ) ;
#17970=DIRECTION ( 'NONE',  ( 0.000000000000000000, 0.000000000000000000, 1.000000000000000000 ) ) ;
#18028=CARTESIAN_POINT ( 'NONE',  ( 0.000000000000000000, 0.000000000000000000, 0.000000000000000000 ) ) ;
#18087=EDGE_LOOP ( 'NONE', ( #2981, #1041 ) ) ;
#18094=ORIENTED_EDGE ( 'NONE', *, *, #2125, .T. ) ;
#18109=DIRECTION ( 'NONE',  ( -0.000000000000000000, -0.000000000000000000, -1.000000000000000000 ) ) ;
#18130=AXIS2_PLACEMENT_3D ( 'NONE', #16065, #7728, #21319 ) ;
#18180=FACE_OUTER_BOUND ( 'NONE', #20289, .T. ) ;
#18207=PLANE ( 'NONE',  #660 ) ;
#18211=CARTESIAN_POINT ( 'NONE',  ( 0.000000000000000000, 0.000000000000000000, -65.00000000000000000 ) ) ;
#18220=DIRECTION ( 'NONE',  ( -1.000000000000000000, 0.000000000000000000, -0.000000000000000000 ) ) ;
#18270=AXIS2_PLACEMENT_3D ( 'NONE', #18534, #1534, #22129 ) ;
#18313=CARTESIAN_POINT ( 'NONE',  ( 1.322875655532295358, 1.500000000000000000, -378.2244600276337678 ) ) ;
#18314=EDGE_LOOP ( 'NONE', ( #9096, #6748, #9360, #20921 ) ) ;
#18319=CARTESIAN_POINT ( 'NONE',  ( -21.50000000000001066, 0.000000000000000000, -30.00000000000000000 ) ) ;
#18432=AXIS2_PLACEMENT_3D ( 'NONE', #14230, #17822, #12304 ) ;
#18534=CARTESIAN_POINT ( 'NONE',  ( 0.000000000000000000, 0.000000000000000000, -55.00000000000000711 ) ) ;
#18542=CARTESIAN_POINT ( 'NONE',  ( 0.000000000000000000, 0.000000000000000000, -120.0000000000000142 ) ) ;
#18546=EDGE_CURVE ( 'NONE', #9212, #16736, #6194, .T. ) ;
#18605=EDGE_LOOP ( 'NONE', ( #6669, #15416, #7612, #4592 ) ) ;
#18650=VERTEX_POINT ( 'NONE', #6524 ) ;
#18653=DIRECTION ( 'NONE',  ( 0.000000000000000000, 0.000000000000000000, 1.000000000000000000 ) ) ;
#18694=SURFACE_STYLE_USAGE ( .BOTH. , #13745 ) ;
#18782=ORIENTED_EDGE ( 'NONE', *, *, #9403, .T. ) ;
#18790=CIRCLE ( 'NONE', #19138, 2.000000000000000000 ) ;
#18884=CIRCLE ( 'NONE', #20287, 2.000000000000000000 ) ;
#18893=ORIENTED_EDGE ( 'NONE', *, *, #9134, .F. ) ;
#19026=DIRECTION ( 'NONE',  ( -1.000000000000000000, 1.224646799147353454E-16, 0.000000000000000000 ) ) ;
#19049=CARTESIAN_POINT ( 'NONE',  ( -2.000000000000000000, 2.449293598294706414E-16, -70.00000000000000000 ) ) ;
#19067=DIRECTION ( 'NONE',  ( -0.000000000000000000, -0.000000000000000000, -1.000000000000000000 ) ) ;
#19099=ORIENTED_EDGE ( 'NONE', *, *, #22019, .T. ) ;
#19110=AXIS2_PLACEMENT_3D ( 'NONE', #11787, #18653, #3214 ) ;
#19138=AXIS2_PLACEMENT_3D ( 'NONE', #10066, #8385, #22099 ) ;
#19229=DIRECTION ( 'NONE',  ( 1.000000000000000000, 0.000000000000000000, 0.000000000000000000 ) ) ;
#19239=EDGE_LOOP ( 'NONE', ( #13295, #1889, #7942, #20418 ) ) ;
#19241=ORIENTED_EDGE ( 'NONE', *, *, #17683, .T. ) ;
#19248=FACE_OUTER_BOUND ( 'NONE', #3879, .T. ) ;
#19264=SURFACE_SIDE_STYLE ('',( #20946 ) ) ;
#19369=CARTESIAN_POINT ( 'NONE',  ( 1.322875655532295136, 1.500000000000000000, -120.0000000000000142 ) ) ;
#19408=LINE ( 'NONE', #2307, #2932 ) ;
#19422=PLANE ( 'NONE',  #1544 ) ;
#19514=DIRECTION ( 'NONE',  ( 0.000000000000000000, 0.000000000000000000, 1.000000000000000000 ) ) ;
#19521=SHAPE_DEFINITION_REPRESENTATION ( #8534, #21505 ) ;
#19535=LINE ( 'NONE', #20890, #13050 ) ;
#19566=ORIENTED_EDGE ( 'NONE', *, *, #1509, .T. ) ;
#19588=LINE ( 'NONE', #17481, #7414 ) ;
#19638=CARTESIAN_POINT ( 'NONE',  ( 0.000000000000000000, 0.000000000000000000, -65.00000000000000000 ) ) ;
#19653=CARTESIAN_POINT ( 'NONE',  ( 12.50000000000000355, 0.000000000000000000, -25.00000000000000000 ) ) ;
#19755=ORIENTED_EDGE ( 'NONE', *, *, #15025, .T. ) ;
#19790=EDGE_CURVE ( 'NONE', #10050, #21036, #120, .T. ) ;
#19811=CARTESIAN_POINT ( 'NONE',  ( 17.50000000000000355, 0.000000000000000000, -65.00000000000000000 ) ) ;
#19926=DIRECTION ( 'NONE',  ( -1.000000000000000000, 0.000000000000000000, 0.000000000000000000 ) ) ;
#20015=ADVANCED_FACE ( 'NONE', ( #11568 ), #10416, .T. ) ;
#20131=FILL_AREA_STYLE_COLOUR ( '', #14239 ) ;
#20154=DIRECTION ( 'NONE',  ( -0.000000000000000000, -0.000000000000000000, -1.000000000000000000 ) ) ;
#20188=ORIENTED_EDGE ( 'NONE', *, *, #17171, .T. ) ;
#20200=UNCERTAINTY_MEASURE_WITH_UNIT (LENGTH_MEASURE( 1.000000000000000082E-05 ), #12296, 'distance_accuracy_value', 'NONE');
#20287=AXIS2_PLACEMENT_3D ( 'NONE', #4354, #18109, #5833 ) ;
#20289=EDGE_LOOP ( 'NONE', ( #2624, #19099 ) ) ;
#20347=PRODUCT_DEFINITION_FORMATION_WITH_SPECIFIED_SOURCE ( 'ANY', '', #20542, .NOT_KNOWN. ) ;
#20358=EDGE_CURVE ( 'NONE', #16402, #3040, #8735, .T. ) ;
#20359=SURFACE_STYLE_FILL_AREA ( #20582 ) ;
#20408=DIRECTION ( 'NONE',  ( 1.224646799147353207E-16, 1.000000000000000000, -0.000000000000000000 ) ) ;
#20418=ORIENTED_EDGE ( 'NONE', *, *, #11174, .T. ) ;
#20526=CIRCLE ( 'NONE', #16591, 17.50000000000000355 ) ;
#20542=PRODUCT ( 'motor', 'motor', '', ( #12673 ) ) ;
#20582=FILL_AREA_STYLE ('',( #20131 ) ) ;
#20629=ORIENTED_EDGE ( 'NONE', *, *, #10180, .F. ) ;
#20674=VERTEX_POINT ( 'NONE', #9178 ) ;
#20689=AXIS2_PLACEMENT_3D ( 'NONE', #3510, #10390, #10610 ) ;
#20705=AXIS2_PLACEMENT_3D ( 'NONE', #4838, #11714, #10556 ) ;
#20742=ORIENTED_EDGE ( 'NONE', *, *, #12429, .T. ) ;
#20890=CARTESIAN_POINT ( 'NONE',  ( -2.000000000000000000, 2.449293598294706414E-16, -120.0000000000000142 ) ) ;
#20906=CIRCLE ( 'NONE', #17676, 21.50000000000001066 ) ;
#20909=AXIS2_PLACEMENT_3D ( 'NONE', #11250, #2575, #14744 ) ;
#20921=ORIENTED_EDGE ( 'NONE', *, *, #6066, .F. ) ;
#20923=ORIENTED_EDGE ( 'NONE', *, *, #18546, .F. ) ;
#20946=SURFACE_STYLE_FILL_AREA ( #12412 ) ;
#21015=DIRECTION ( 'NONE',  ( 1.000000000000000000, 0.000000000000000000, 0.000000000000000000 ) ) ;
#21036=VERTEX_POINT ( 'NONE', #21083 ) ;
#21054=DIRECTION ( 'NONE',  ( -1.000000000000000000, 0.000000000000000000, 0.000000000000000000 ) ) ;
#21065=LINE ( 'NONE', #4185, #13398 ) ;
#21072=EDGE_CURVE ( 'NONE', #21666, #21036, #4302, .T. ) ;
#21083=CARTESIAN_POINT ( 'NONE',  ( 21.50000000000000711, 2.632990618166810418E-15, -55.00000000000000711 ) ) ;
#21092=ADVANCED_FACE ( 'NONE', ( #1275 ), #14903, .T. ) ;
#21149=DIRECTION ( 'NONE',  ( 1.000000000000000000, 0.000000000000000000, -0.000000000000000000 ) ) ;
#21319=DIRECTION ( 'NONE',  ( 1.000000000000000000, 0.000000000000000000, 0.000000000000000000 ) ) ;
#21323=DIRECTION ( 'NONE',  ( 0.000000000000000000, 0.000000000000000000, 1.000000000000000000 ) ) ;
#21505=SHAPE_REPRESENTATION ( 'motor', ( #6677 ), #1652 ) ;
#21548=DIRECTION ( 'NONE',  ( -1.000000000000000000, 0.000000000000000000, 0.000000000000000000 ) ) ;
#21574=CARTESIAN_POINT ( 'NONE',  ( 0.000000000000000000, 0.000000000000000000, -25.00000000000000000 ) ) ;
#21653=CARTESIAN_POINT ( 'NONE',  ( 17.50000000000001066, 0.000000000000000000, -30.00000000000000000 ) ) ;
#21666=VERTEX_POINT ( 'NONE', #13551 ) ;
#21684=PLANE ( 'NONE',  #10927 ) ;
#21735=ORIENTED_EDGE ( 'NONE', *, *, #18546, .T. ) ;
#21744=CARTESIAN_POINT ( 'NONE',  ( 0.000000000000000000, 0.000000000000000000, -70.00000000000000000 ) ) ;
#21759=STYLED_ITEM ( 'NONE', ( #10724 ), #22038 ) ;
#21763=ORIENTED_EDGE ( 'NONE', *, *, #17120, .F. ) ;
#21824=CARTESIAN_POINT ( 'NONE',  ( 0.000000000000000000, 0.000000000000000000, -120.0000000000000142 ) ) ;
#21845=ADVANCED_FACE ( 'NONE', ( #8598 ), #12079, .T. ) ;
#21888=EDGE_CURVE ( 'NONE', #9986, #16736, #19588, .T. ) ;
#21893=CARTESIAN_POINT ( 'NONE',  ( 0.000000000000000000, 0.000000000000000000, -25.00000000000000000 ) ) ;
#22019=EDGE_CURVE ( 'NONE', #21036, #10050, #1289, .T. ) ;
#22038=MANIFOLD_SOLID_BREP ( 'Revolve1', #12174 ) ;
#22099=DIRECTION ( 'NONE',  ( -1.000000000000000000, 0.000000000000000000, 0.000000000000000000 ) ) ;
#22129=DIRECTION ( 'NONE',  ( -1.000000000000000000, 0.000000000000000000, 0.000000000000000000 ) ) ;
#22237=FACE_OUTER_BOUND ( 'NONE', #3153, .T. ) ;
ENDSEC;
END-ISO-10303-21;
